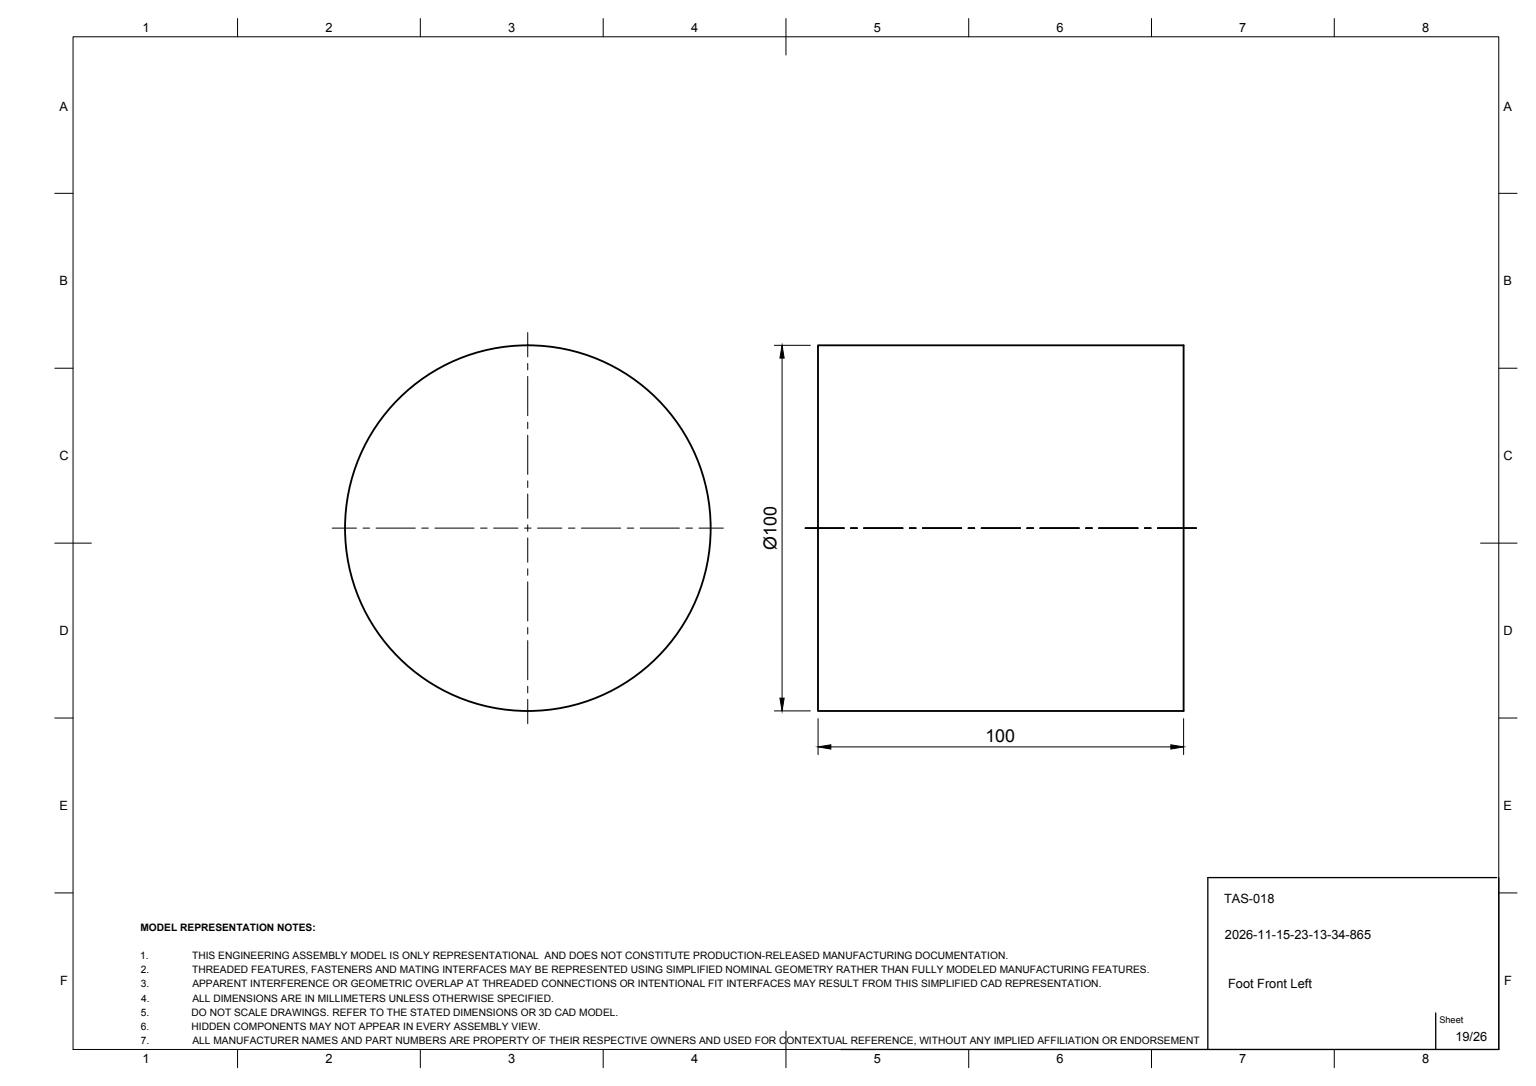
ISO-10303-21;
HEADER;
/* Generated by software containing ST-Developer
 * from STEP Tools, Inc. (www.steptools.com) 
 */

FILE_DESCRIPTION(
/* description */ (''),
/* implementation_level */ '2;1');

FILE_NAME(
/* name */ 'Foot Front Left.step',
/* time_stamp */ '2026-11-15T15:17:57-08:00',
/* author */ (''),
/* organization */ (''),
/* preprocessor_version */ 'ST-DEVELOPER v20.2',
/* originating_system */ 'Autodesk Translation Framework v15.17.0.0',
/* authorisation */ '');

FILE_SCHEMA (('AUTOMOTIVE_DESIGN { 1 0 10303 214 3 1 1 }'));
ENDSEC;

DATA;
#10=MECHANICAL_DESIGN_GEOMETRIC_PRESENTATION_REPRESENTATION('',(#194),#3723);
#15=CIRCLE('',#2436,1.96850393700787);
#16=CIRCLE('',#2437,1.96850393700787);
#25=CYLINDRICAL_SURFACE('',#2435,1.96850393700787);
#146=SHAPE_REPRESENTATION_RELATIONSHIP('SRR','None',#3827,#170);
#170=ADVANCED_BREP_SHAPE_REPRESENTATION('',(#218),#3716);
#194=STYLED_ITEM('',(#3945),#218);
#218=MANIFOLD_SOLID_BREP('Body1',#2042);
#321=FACE_OUTER_BOUND('',#447,.T.);
#322=FACE_OUTER_BOUND('',#448,.T.);
#323=FACE_OUTER_BOUND('',#449,.T.);
#447=EDGE_LOOP('',(#1683,#1684,#1685,#1686));
#448=EDGE_LOOP('',(#1687));
#449=EDGE_LOOP('',(#1688));
#659=LINE('',#3534,#881);
#881=VECTOR('',#2931,1.96850393700787);
#1045=VERTEX_POINT('',#3531);
#1046=VERTEX_POINT('',#3533);
#1263=EDGE_CURVE('',#1045,#1045,#15,.T.);
#1264=EDGE_CURVE('',#1045,#1046,#659,.T.);
#1265=EDGE_CURVE('',#1046,#1046,#16,.T.);
#1683=ORIENTED_EDGE('',*,*,#1263,.T.);
#1684=ORIENTED_EDGE('',*,*,#1264,.T.);
#1685=ORIENTED_EDGE('',*,*,#1265,.F.);
#1686=ORIENTED_EDGE('',*,*,#1264,.F.);
#1687=ORIENTED_EDGE('',*,*,#1265,.T.);
#1688=ORIENTED_EDGE('',*,*,#1263,.F.);
#1873=PLANE('',#2438);
#1874=PLANE('',#2439);
#1995=ADVANCED_FACE('',(#321),#25,.T.);
#1996=ADVANCED_FACE('',(#322),#1873,.T.);
#1997=ADVANCED_FACE('',(#323),#1874,.F.);
#2042=CLOSED_SHELL('',(#1995,#1996,#1997));
#2434=AXIS2_PLACEMENT_3D('',#3529,#2925,#2926);
#2435=AXIS2_PLACEMENT_3D('',#3530,#2927,#2928);
#2436=AXIS2_PLACEMENT_3D('',#3532,#2929,#2930);
#2437=AXIS2_PLACEMENT_3D('',#3535,#2932,#2933);
#2438=AXIS2_PLACEMENT_3D('',#3536,#2934,#2935);
#2439=AXIS2_PLACEMENT_3D('',#3537,#2936,#2937);
#2925=DIRECTION('axis',(0.,0.,1.));
#2926=DIRECTION('refdir',(1.,0.,0.));
#2927=DIRECTION('center_axis',(0.,1.,0.));
#2928=DIRECTION('ref_axis',(0.,0.,1.));
#2929=DIRECTION('center_axis',(0.,-1.,0.));
#2930=DIRECTION('ref_axis',(0.,0.,-1.));
#2931=DIRECTION('',(0.,-1.,0.));
#2932=DIRECTION('center_axis',(0.,-1.,0.));
#2933=DIRECTION('ref_axis',(0.,0.,-1.));
#2934=DIRECTION('center_axis',(0.,-1.,0.));
#2935=DIRECTION('ref_axis',(0.,0.,-1.));
#2936=DIRECTION('center_axis',(0.,-1.,0.));
#2937=DIRECTION('ref_axis',(0.,0.,-1.));
#3529=CARTESIAN_POINT('',(0.,0.,0.));
#3530=CARTESIAN_POINT('Origin',(-33.6377952755905,-4.91732638859567E-15,
19.6377952755906));
#3531=CARTESIAN_POINT('',(-33.6377952755905,3.93700787401574,17.6692913385827));
#3532=CARTESIAN_POINT('Origin',(-33.6377952755905,3.93700787401574,19.6377952755906));
#3533=CARTESIAN_POINT('',(-33.6377952755905,-4.91732638859567E-15,17.6692913385827));
#3534=CARTESIAN_POINT('',(-33.6377952755905,-4.91732638859567E-15,17.6692913385827));
#3535=CARTESIAN_POINT('Origin',(-33.6377952755905,-4.91732638859567E-15,
19.6377952755906));
#3536=CARTESIAN_POINT('Origin',(-33.6377952755905,-4.91732638859567E-15,
19.6377952755906));
#3537=CARTESIAN_POINT('Origin',(-33.6377952755905,3.93700787401574,19.6377952755906));
#3689=UNCERTAINTY_MEASURE_WITH_UNIT(LENGTH_MEASURE(0.000393700787401575),
#3725,'DISTANCE_ACCURACY_VALUE',
'Maximum model space distance between geometric entities at asserted c
onnectivities');
#3696=UNCERTAINTY_MEASURE_WITH_UNIT(LENGTH_MEASURE(0.000393700787401575),
#3725,'DISTANCE_ACCURACY_VALUE',
'Maximum model space distance between geometric entities at asserted c
onnectivities');
#3716=(
GEOMETRIC_REPRESENTATION_CONTEXT(3)
GLOBAL_UNCERTAINTY_ASSIGNED_CONTEXT((#3689))
GLOBAL_UNIT_ASSIGNED_CONTEXT((#3725,#3729,#3730))
REPRESENTATION_CONTEXT('','3D')
);
#3723=(
GEOMETRIC_REPRESENTATION_CONTEXT(3)
GLOBAL_UNCERTAINTY_ASSIGNED_CONTEXT((#3696))
GLOBAL_UNIT_ASSIGNED_CONTEXT((#3725,#3729,#3730))
REPRESENTATION_CONTEXT('','3D')
);
#3724=DIMENSIONAL_EXPONENTS(1.,0.,0.,0.,0.,0.,0.);
#3725=(
CONVERSION_BASED_UNIT('inch',#3728)
LENGTH_UNIT()
NAMED_UNIT(#3724)
);
#3726=(
LENGTH_UNIT()
NAMED_UNIT(*)
SI_UNIT(.MILLI.,.METRE.)
);
#3728=LENGTH_MEASURE_WITH_UNIT(LENGTH_MEASURE(25.4),#3726);
#3729=(
NAMED_UNIT(*)
PLANE_ANGLE_UNIT()
SI_UNIT($,.RADIAN.)
);
#3730=(
NAMED_UNIT(*)
SI_UNIT($,.STERADIAN.)
SOLID_ANGLE_UNIT()
);
#3750=SHAPE_DEFINITION_REPRESENTATION(#3777,#3827);
#3777=PRODUCT_DEFINITION_SHAPE('',$,#3854);
#3827=SHAPE_REPRESENTATION('',(#2434),#3716);
#3834=PRODUCT_DEFINITION_CONTEXT('part definition',#3914,'design');
#3854=PRODUCT_DEFINITION('2026-11-15-23-13-34-865','Foot Front Left',#3880,
#3834);
#3880=PRODUCT_DEFINITION_FORMATION('',$,#3935);
#3914=APPLICATION_CONTEXT(
'Core Data for Automotive Mechanical Design Process');
#3915=PRODUCT_CONTEXT('part definition',#3914,'mechanical');
#3935=PRODUCT('2026-11-15-23-13-34-865','Foot Front Left',$,(#3915));
#3945=PRESENTATION_STYLE_ASSIGNMENT((#3953));
#3953=SURFACE_STYLE_USAGE(.BOTH.,#3961);
#3961=SURFACE_SIDE_STYLE('',(#3969));
#3969=SURFACE_STYLE_FILL_AREA(#3977);
#3977=FILL_AREA_STYLE('Black',(#3985));
#3985=FILL_AREA_STYLE_COLOUR('Black',#3993);
#3993=COLOUR_RGB('Black',0.0784313725490196,0.0784313725490196,0.0784313725490196);
ENDSEC;
END-ISO-10303-21;
